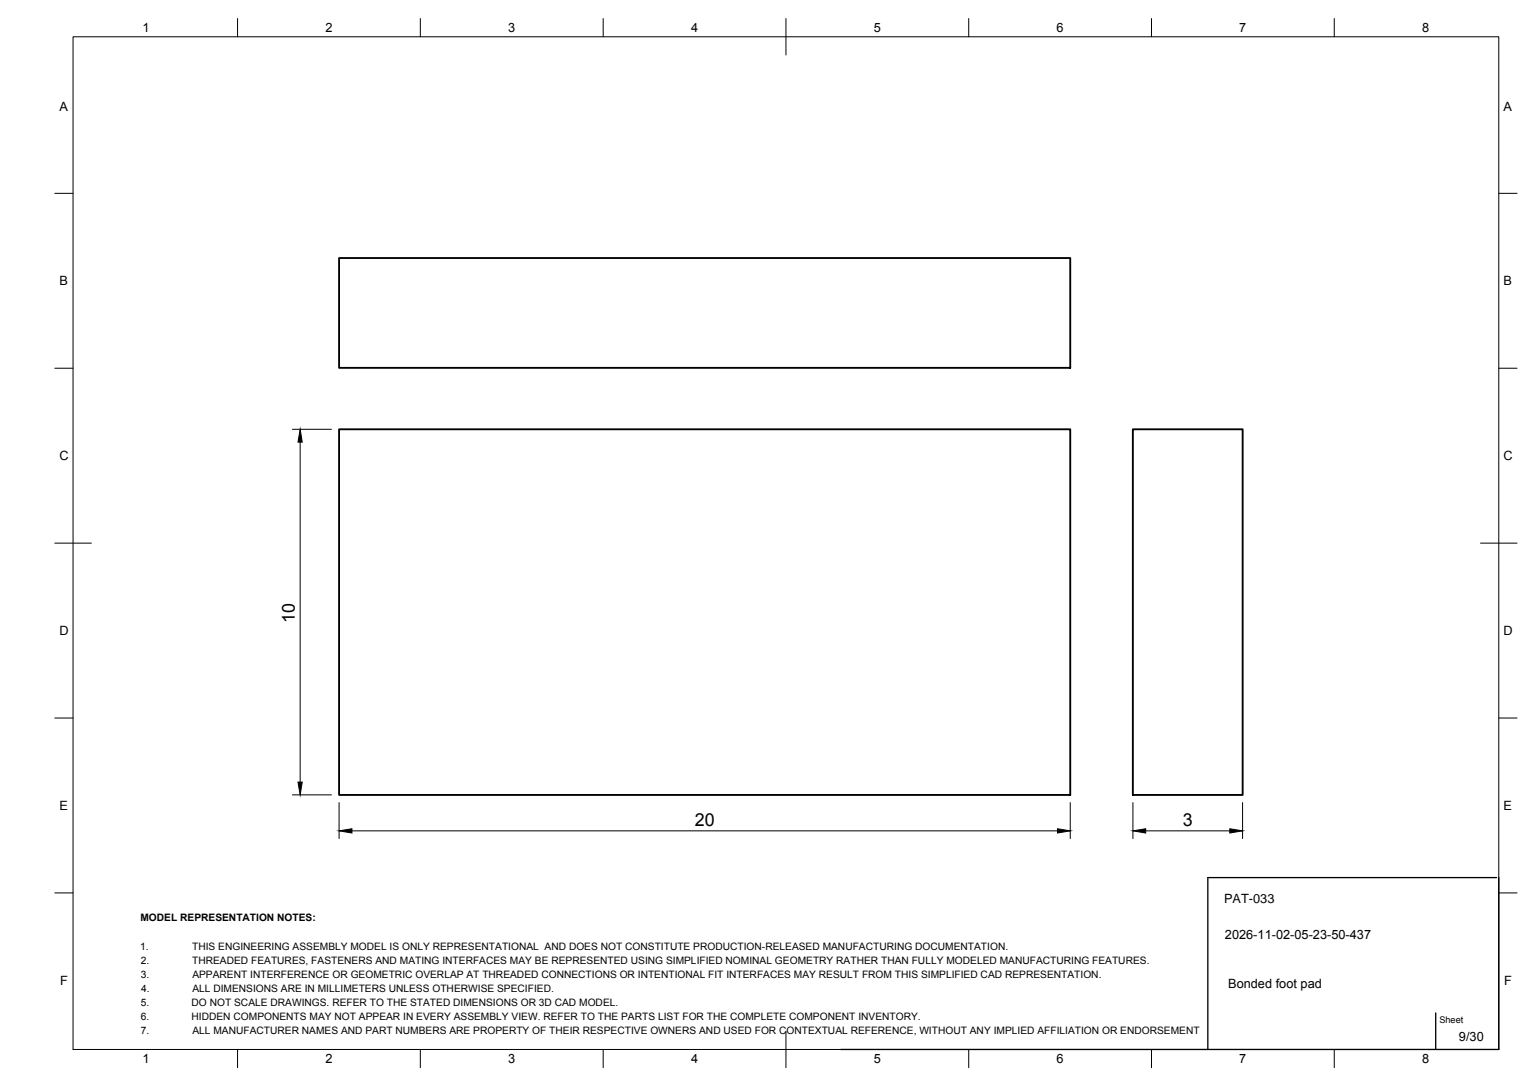
ISO-10303-21;
HEADER;
/* Generated by software containing ST-Developer
 * from STEP Tools, Inc. (www.steptools.com) 
 */

FILE_DESCRIPTION(
/* description */ ('Dual-rail gantry carriage'),
/* implementation_level */ '2;1');

FILE_NAME(
/* name */ 'Bonded foot pad.step',
/* time_stamp */ '2026-10-27T10:49:15-07:00',
/* author */ (''),
/* organization */ (''),
/* preprocessor_version */ 'ST-DEVELOPER v20.2',
/* originating_system */ 'Autodesk Translation Framework v15.17.0.0',
/* authorisation */ '');

FILE_SCHEMA (('AUTOMOTIVE_DESIGN { 1 0 10303 214 3 1 1 }'));
ENDSEC;

DATA;
#10=MECHANICAL_DESIGN_GEOMETRIC_PRESENTATION_REPRESENTATION('',(#589),#12804);
#527=SHAPE_REPRESENTATION_RELATIONSHIP('SRR','None',#13005,#558);
#558=ADVANCED_BREP_SHAPE_REPRESENTATION('',(#620),#12775);
#589=STYLED_ITEM('',(#13240),#620);
#620=MANIFOLD_SOLID_BREP('Body1',#7367);
#788=PLANE('',#7820);
#789=PLANE('',#7821);
#790=PLANE('',#7822);
#791=PLANE('',#7823);
#792=PLANE('',#7824);
#793=PLANE('',#7825);
#1088=FACE_OUTER_BOUND('',#1509,.T.);
#1089=FACE_OUTER_BOUND('',#1510,.T.);
#1090=FACE_OUTER_BOUND('',#1511,.T.);
#1091=FACE_OUTER_BOUND('',#1512,.T.);
#1092=FACE_OUTER_BOUND('',#1513,.T.);
#1093=FACE_OUTER_BOUND('',#1514,.T.);
#1509=EDGE_LOOP('',(#5259,#5260,#5261,#5262));
#1510=EDGE_LOOP('',(#5263,#5264,#5265,#5266));
#1511=EDGE_LOOP('',(#5267,#5268,#5269,#5270));
#1512=EDGE_LOOP('',(#5271,#5272,#5273,#5274));
#1513=EDGE_LOOP('',(#5275,#5276,#5277,#5278));
#1514=EDGE_LOOP('',(#5279,#5280,#5281,#5282));
#2012=LINE('',#10898,#2721);
#2013=LINE('',#10900,#2722);
#2014=LINE('',#10902,#2723);
#2015=LINE('',#10903,#2724);
#2016=LINE('',#10906,#2725);
#2017=LINE('',#10908,#2726);
#2018=LINE('',#10909,#2727);
#2019=LINE('',#10912,#2728);
#2020=LINE('',#10914,#2729);
#2021=LINE('',#10915,#2730);
#2022=LINE('',#10917,#2731);
#2023=LINE('',#10918,#2732);
#2721=VECTOR('',#8711,1.);
#2722=VECTOR('',#8712,1.);
#2723=VECTOR('',#8713,1.);
#2724=VECTOR('',#8714,1.);
#2725=VECTOR('',#8717,1.);
#2726=VECTOR('',#8718,1.);
#2727=VECTOR('',#8719,1.);
#2728=VECTOR('',#8722,1.);
#2729=VECTOR('',#8723,1.);
#2730=VECTOR('',#8724,1.);
#2731=VECTOR('',#8727,1.);
#2732=VECTOR('',#8728,1.);
#3630=VERTEX_POINT('',#10896);
#3631=VERTEX_POINT('',#10897);
#3632=VERTEX_POINT('',#10899);
#3633=VERTEX_POINT('',#10901);
#3634=VERTEX_POINT('',#10905);
#3635=VERTEX_POINT('',#10907);
#3636=VERTEX_POINT('',#10911);
#3637=VERTEX_POINT('',#10913);
#4252=EDGE_CURVE('',#3630,#3631,#2012,.T.);
#4253=EDGE_CURVE('',#3631,#3632,#2013,.T.);
#4254=EDGE_CURVE('',#3633,#3632,#2014,.T.);
#4255=EDGE_CURVE('',#3630,#3633,#2015,.T.);
#4256=EDGE_CURVE('',#3634,#3630,#2016,.T.);
#4257=EDGE_CURVE('',#3635,#3633,#2017,.T.);
#4258=EDGE_CURVE('',#3634,#3635,#2018,.T.);
#4259=EDGE_CURVE('',#3636,#3634,#2019,.T.);
#4260=EDGE_CURVE('',#3637,#3635,#2020,.T.);
#4261=EDGE_CURVE('',#3636,#3637,#2021,.T.);
#4262=EDGE_CURVE('',#3631,#3636,#2022,.T.);
#4263=EDGE_CURVE('',#3632,#3637,#2023,.T.);
#5259=ORIENTED_EDGE('',*,*,#4252,.T.);
#5260=ORIENTED_EDGE('',*,*,#4253,.T.);
#5261=ORIENTED_EDGE('',*,*,#4254,.F.);
#5262=ORIENTED_EDGE('',*,*,#4255,.F.);
#5263=ORIENTED_EDGE('',*,*,#4256,.T.);
#5264=ORIENTED_EDGE('',*,*,#4255,.T.);
#5265=ORIENTED_EDGE('',*,*,#4257,.F.);
#5266=ORIENTED_EDGE('',*,*,#4258,.F.);
#5267=ORIENTED_EDGE('',*,*,#4259,.T.);
#5268=ORIENTED_EDGE('',*,*,#4258,.T.);
#5269=ORIENTED_EDGE('',*,*,#4260,.F.);
#5270=ORIENTED_EDGE('',*,*,#4261,.F.);
#5271=ORIENTED_EDGE('',*,*,#4262,.T.);
#5272=ORIENTED_EDGE('',*,*,#4261,.T.);
#5273=ORIENTED_EDGE('',*,*,#4263,.F.);
#5274=ORIENTED_EDGE('',*,*,#4253,.F.);
#5275=ORIENTED_EDGE('',*,*,#4263,.T.);
#5276=ORIENTED_EDGE('',*,*,#4260,.T.);
#5277=ORIENTED_EDGE('',*,*,#4257,.T.);
#5278=ORIENTED_EDGE('',*,*,#4254,.T.);
#5279=ORIENTED_EDGE('',*,*,#4262,.F.);
#5280=ORIENTED_EDGE('',*,*,#4252,.F.);
#5281=ORIENTED_EDGE('',*,*,#4256,.F.);
#5282=ORIENTED_EDGE('',*,*,#4259,.F.);
#7014=ADVANCED_FACE('',(#1088),#788,.T.);
#7015=ADVANCED_FACE('',(#1089),#789,.T.);
#7016=ADVANCED_FACE('',(#1090),#790,.T.);
#7017=ADVANCED_FACE('',(#1091),#791,.T.);
#7018=ADVANCED_FACE('',(#1092),#792,.T.);
#7019=ADVANCED_FACE('',(#1093),#793,.F.);
#7367=CLOSED_SHELL('',(#7014,#7015,#7016,#7017,#7018,#7019));
#7819=AXIS2_PLACEMENT_3D('',#10894,#8707,#8708);
#7820=AXIS2_PLACEMENT_3D('',#10895,#8709,#8710);
#7821=AXIS2_PLACEMENT_3D('',#10904,#8715,#8716);
#7822=AXIS2_PLACEMENT_3D('',#10910,#8720,#8721);
#7823=AXIS2_PLACEMENT_3D('',#10916,#8725,#8726);
#7824=AXIS2_PLACEMENT_3D('',#10919,#8729,#8730);
#7825=AXIS2_PLACEMENT_3D('',#10920,#8731,#8732);
#8707=DIRECTION('axis',(0.,0.,1.));
#8708=DIRECTION('refdir',(1.,0.,0.));
#8709=DIRECTION('center_axis',(0.,1.,0.));
#8710=DIRECTION('ref_axis',(-1.,0.,0.));
#8711=DIRECTION('',(-1.,0.,0.));
#8712=DIRECTION('',(0.,0.,1.));
#8713=DIRECTION('',(-1.,0.,0.));
#8714=DIRECTION('',(0.,0.,1.));
#8715=DIRECTION('center_axis',(1.,0.,0.));
#8716=DIRECTION('ref_axis',(0.,1.,0.));
#8717=DIRECTION('',(0.,1.,0.));
#8718=DIRECTION('',(0.,1.,0.));
#8719=DIRECTION('',(0.,0.,1.));
#8720=DIRECTION('center_axis',(0.,-1.,0.));
#8721=DIRECTION('ref_axis',(1.,0.,0.));
#8722=DIRECTION('',(1.,0.,0.));
#8723=DIRECTION('',(1.,0.,0.));
#8724=DIRECTION('',(0.,0.,1.));
#8725=DIRECTION('center_axis',(-1.,0.,0.));
#8726=DIRECTION('ref_axis',(0.,-1.,0.));
#8727=DIRECTION('',(0.,-1.,0.));
#8728=DIRECTION('',(0.,-1.,0.));
#8729=DIRECTION('center_axis',(0.,0.,1.));
#8730=DIRECTION('ref_axis',(1.,0.,0.));
#8731=DIRECTION('center_axis',(0.,0.,1.));
#8732=DIRECTION('ref_axis',(1.,0.,0.));
#10894=CARTESIAN_POINT('',(0.,0.,0.));
#10895=CARTESIAN_POINT('Origin',(2.,-11.5,-1.1));
#10896=CARTESIAN_POINT('',(2.,-11.5,-1.1));
#10897=CARTESIAN_POINT('',(0.,-11.5,-1.1));
#10898=CARTESIAN_POINT('',(2.,-11.5,-1.1));
#10899=CARTESIAN_POINT('',(0.,-11.5,-0.8));
#10900=CARTESIAN_POINT('',(0.,-11.5,-1.1));
#10901=CARTESIAN_POINT('',(2.,-11.5,-0.8));
#10902=CARTESIAN_POINT('',(2.,-11.5,-0.8));
#10903=CARTESIAN_POINT('',(2.,-11.5,-1.1));
#10904=CARTESIAN_POINT('Origin',(2.,-12.5,-1.1));
#10905=CARTESIAN_POINT('',(2.,-12.5,-1.1));
#10906=CARTESIAN_POINT('',(2.,-12.5,-1.1));
#10907=CARTESIAN_POINT('',(2.,-12.5,-0.8));
#10908=CARTESIAN_POINT('',(2.,-12.5,-0.8));
#10909=CARTESIAN_POINT('',(2.,-12.5,-1.1));
#10910=CARTESIAN_POINT('Origin',(0.,-12.5,-1.1));
#10911=CARTESIAN_POINT('',(0.,-12.5,-1.1));
#10912=CARTESIAN_POINT('',(0.,-12.5,-1.1));
#10913=CARTESIAN_POINT('',(0.,-12.5,-0.8));
#10914=CARTESIAN_POINT('',(0.,-12.5,-0.8));
#10915=CARTESIAN_POINT('',(0.,-12.5,-1.1));
#10916=CARTESIAN_POINT('Origin',(0.,-11.5,-1.1));
#10917=CARTESIAN_POINT('',(0.,-11.5,-1.1));
#10918=CARTESIAN_POINT('',(0.,-11.5,-0.8));
#10919=CARTESIAN_POINT('Origin',(1.,-12.,-0.8));
#10920=CARTESIAN_POINT('Origin',(1.,-12.,-1.1));
#12739=UNCERTAINTY_MEASURE_WITH_UNIT(LENGTH_MEASURE(0.001),#12805,
'DISTANCE_ACCURACY_VALUE',
'Maximum model space distance between geometric entities at asserted c
onnectivities');
#12768=UNCERTAINTY_MEASURE_WITH_UNIT(LENGTH_MEASURE(0.001),#12805,
'DISTANCE_ACCURACY_VALUE',
'Maximum model space distance between geometric entities at asserted c
onnectivities');
#12775=(
GEOMETRIC_REPRESENTATION_CONTEXT(3)
GLOBAL_UNCERTAINTY_ASSIGNED_CONTEXT((#12739))
GLOBAL_UNIT_ASSIGNED_CONTEXT((#12805,#12807,#12808))
REPRESENTATION_CONTEXT('','3D')
);
#12804=(
GEOMETRIC_REPRESENTATION_CONTEXT(3)
GLOBAL_UNCERTAINTY_ASSIGNED_CONTEXT((#12768))
GLOBAL_UNIT_ASSIGNED_CONTEXT((#12805,#12807,#12808))
REPRESENTATION_CONTEXT('','3D')
);
#12805=(
LENGTH_UNIT()
NAMED_UNIT(*)
SI_UNIT(.CENTI.,.METRE.)
);
#12807=(
NAMED_UNIT(*)
PLANE_ANGLE_UNIT()
SI_UNIT($,.RADIAN.)
);
#12808=(
NAMED_UNIT(*)
SI_UNIT($,.STERADIAN.)
SOLID_ANGLE_UNIT()
);
#12815=SHAPE_DEFINITION_REPRESENTATION(#12850,#13005);
#12850=PRODUCT_DEFINITION_SHAPE('',$,#13041);
#13005=SHAPE_REPRESENTATION('',(#7819),#12775);
#13034=PRODUCT_DEFINITION_CONTEXT('part definition',#13141,'design');
#13041=PRODUCT_DEFINITION('Bonded foot pad','Bonded foot pad',#13076,#13034);
#13076=PRODUCT_DEFINITION_FORMATION('',$,#13149);
#13141=APPLICATION_CONTEXT(
'Core Data for Automotive Mechanical Design Process');
#13142=PRODUCT_CONTEXT('part definition',#13141,'mechanical');
#13149=PRODUCT('Bonded foot pad','Bonded foot pad','Bonded foot pad',(#13142));
#13234=COLOUR_RGB('Sky Blue',0.24,0.69,0.87);
#13235=FILL_AREA_STYLE_COLOUR('',#13234);
#13236=FILL_AREA_STYLE('',(#13235));
#13237=SURFACE_STYLE_FILL_AREA(#13236);
#13238=SURFACE_SIDE_STYLE('',(#13237));
#13239=SURFACE_STYLE_USAGE(.BOTH.,#13238);
#13240=PRESENTATION_STYLE_ASSIGNMENT((#13239));
ENDSEC;
END-ISO-10303-21;
